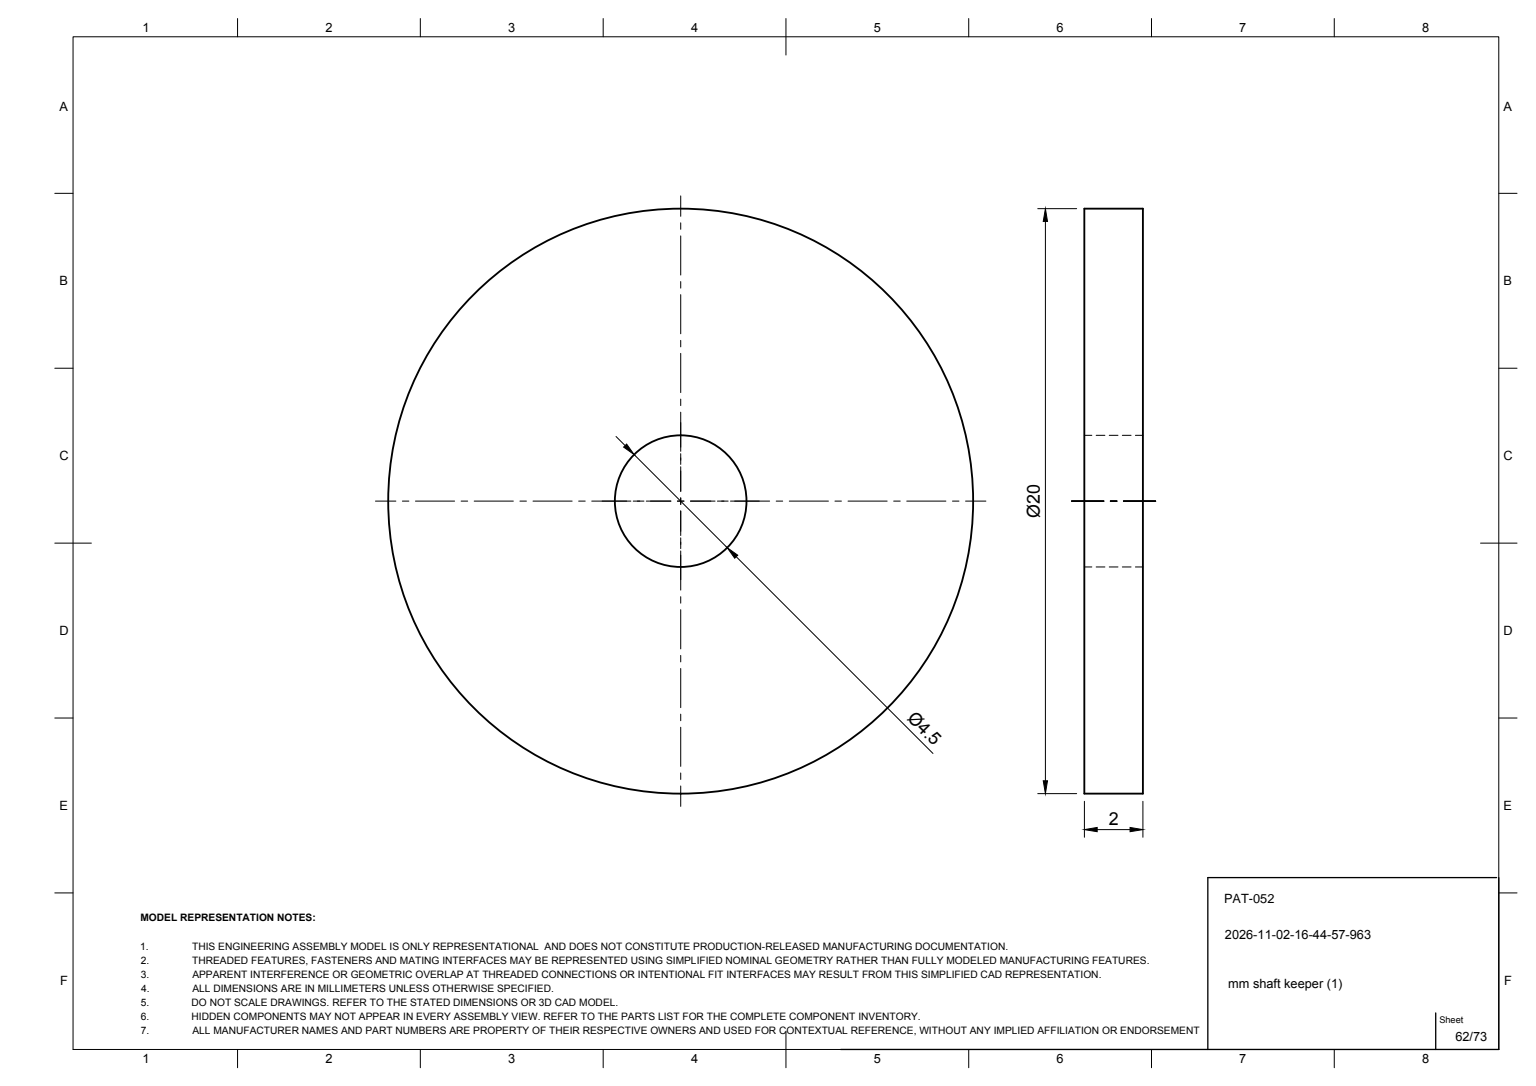
ISO-10303-21;
HEADER;
/* Generated by software containing ST-Developer
 * from STEP Tools, Inc. (www.steptools.com) 
 */

FILE_DESCRIPTION(
/* description */ ('Hand-crank gear train demonstrator'),
/* implementation_level */ '2;1');

FILE_NAME(
/* name */ 'mm shaft keeper (1).step',
/* time_stamp */ '2026-10-28T03:22:13-07:00',
/* author */ (''),
/* organization */ (''),
/* preprocessor_version */ 'ST-DEVELOPER v20.2',
/* originating_system */ 'Autodesk Translation Framework v15.17.0.0',
/* authorisation */ '');

FILE_SCHEMA (('AUTOMOTIVE_DESIGN { 1 0 10303 214 3 1 1 }'));
ENDSEC;

DATA;
#10=MECHANICAL_DESIGN_GEOMETRIC_PRESENTATION_REPRESENTATION('',(#1252),#62758);
#1109=SHAPE_REPRESENTATION_RELATIONSHIP('SRR','None',#63086,#1173);
#1173=ADVANCED_BREP_SHAPE_REPRESENTATION('',(#1327),#62740);
#1252=STYLED_ITEM('',(#63462),#1327);
#1327=MANIFOLD_SOLID_BREP('Body1',#16436);
#1598=FACE_BOUND('',#3889,.T.);
#1599=FACE_BOUND('',#3891,.T.);
#1975=PLANE('',#18269);
#1976=PLANE('',#18270);
#2694=FACE_OUTER_BOUND('',#3886,.T.);
#2695=FACE_OUTER_BOUND('',#3887,.T.);
#2696=FACE_OUTER_BOUND('',#3888,.T.);
#2697=FACE_OUTER_BOUND('',#3890,.T.);
#3886=EDGE_LOOP('',(#13243,#13244,#13245,#13246));
#3887=EDGE_LOOP('',(#13247,#13248,#13249,#13250));
#3888=EDGE_LOOP('',(#13251));
#3889=EDGE_LOOP('',(#13252));
#3890=EDGE_LOOP('',(#13253));
#3891=EDGE_LOOP('',(#13254));
#4978=LINE('',#26767,#6110);
#4979=LINE('',#26773,#6111);
#6110=VECTOR('',#21737,0.225);
#6111=VECTOR('',#21744,1.);
#7018=CIRCLE('',#18264,0.225);
#7019=CIRCLE('',#18265,0.225);
#7020=CIRCLE('',#18267,1.);
#7021=CIRCLE('',#18268,1.);
#8029=VERTEX_POINT('',#26764);
#8030=VERTEX_POINT('',#26766);
#8031=VERTEX_POINT('',#26770);
#8032=VERTEX_POINT('',#26772);
#9873=EDGE_CURVE('',#8029,#8029,#7018,.T.);
#9874=EDGE_CURVE('',#8029,#8030,#4978,.T.);
#9875=EDGE_CURVE('',#8030,#8030,#7019,.T.);
#9876=EDGE_CURVE('',#8031,#8031,#7020,.T.);
#9877=EDGE_CURVE('',#8031,#8032,#4979,.T.);
#9878=EDGE_CURVE('',#8032,#8032,#7021,.T.);
#13243=ORIENTED_EDGE('',*,*,#9873,.F.);
#13244=ORIENTED_EDGE('',*,*,#9874,.T.);
#13245=ORIENTED_EDGE('',*,*,#9875,.T.);
#13246=ORIENTED_EDGE('',*,*,#9874,.F.);
#13247=ORIENTED_EDGE('',*,*,#9876,.F.);
#13248=ORIENTED_EDGE('',*,*,#9877,.T.);
#13249=ORIENTED_EDGE('',*,*,#9878,.T.);
#13250=ORIENTED_EDGE('',*,*,#9877,.F.);
#13251=ORIENTED_EDGE('',*,*,#9876,.T.);
#13252=ORIENTED_EDGE('',*,*,#9873,.T.);
#13253=ORIENTED_EDGE('',*,*,#9878,.F.);
#13254=ORIENTED_EDGE('',*,*,#9875,.F.);
#15342=CYLINDRICAL_SURFACE('',#18263,0.225);
#15343=CYLINDRICAL_SURFACE('',#18266,1.);
#16004=ADVANCED_FACE('',(#2694),#15342,.F.);
#16005=ADVANCED_FACE('',(#2695),#15343,.T.);
#16006=ADVANCED_FACE('',(#2696,#1598),#1975,.T.);
#16007=ADVANCED_FACE('',(#2697,#1599),#1976,.F.);
#16436=CLOSED_SHELL('',(#16004,#16005,#16006,#16007));
#18262=AXIS2_PLACEMENT_3D('',#26762,#21731,#21732);
#18263=AXIS2_PLACEMENT_3D('',#26763,#21733,#21734);
#18264=AXIS2_PLACEMENT_3D('',#26765,#21735,#21736);
#18265=AXIS2_PLACEMENT_3D('',#26768,#21738,#21739);
#18266=AXIS2_PLACEMENT_3D('',#26769,#21740,#21741);
#18267=AXIS2_PLACEMENT_3D('',#26771,#21742,#21743);
#18268=AXIS2_PLACEMENT_3D('',#26774,#21745,#21746);
#18269=AXIS2_PLACEMENT_3D('',#26775,#21747,#21748);
#18270=AXIS2_PLACEMENT_3D('',#26776,#21749,#21750);
#21731=DIRECTION('axis',(0.,0.,1.));
#21732=DIRECTION('refdir',(1.,0.,0.));
#21733=DIRECTION('center_axis',(0.,1.,0.));
#21734=DIRECTION('ref_axis',(1.,0.,0.));
#21735=DIRECTION('center_axis',(0.,-1.,0.));
#21736=DIRECTION('ref_axis',(1.,0.,0.));
#21737=DIRECTION('',(0.,-1.,0.));
#21738=DIRECTION('center_axis',(0.,-1.,0.));
#21739=DIRECTION('ref_axis',(1.,0.,0.));
#21740=DIRECTION('center_axis',(0.,1.,0.));
#21741=DIRECTION('ref_axis',(1.,0.,0.));
#21742=DIRECTION('center_axis',(0.,1.,0.));
#21743=DIRECTION('ref_axis',(1.,0.,0.));
#21744=DIRECTION('',(0.,-1.,0.));
#21745=DIRECTION('center_axis',(0.,1.,0.));
#21746=DIRECTION('ref_axis',(1.,0.,0.));
#21747=DIRECTION('center_axis',(0.,1.,0.));
#21748=DIRECTION('ref_axis',(1.,0.,0.));
#21749=DIRECTION('center_axis',(0.,1.,0.));
#21750=DIRECTION('ref_axis',(1.,0.,0.));
#26762=CARTESIAN_POINT('',(0.,0.,0.));
#26763=CARTESIAN_POINT('Origin',(12.,3.2,9.));
#26764=CARTESIAN_POINT('',(11.775,3.4,9.));
#26765=CARTESIAN_POINT('Origin',(12.,3.4,9.));
#26766=CARTESIAN_POINT('',(11.775,3.2,9.));
#26767=CARTESIAN_POINT('',(11.775,3.2,9.));
#26768=CARTESIAN_POINT('Origin',(12.,3.2,9.));
#26769=CARTESIAN_POINT('Origin',(12.,3.2,9.));
#26770=CARTESIAN_POINT('',(11.,3.4,9.));
#26771=CARTESIAN_POINT('Origin',(12.,3.4,9.));
#26772=CARTESIAN_POINT('',(11.,3.2,9.));
#26773=CARTESIAN_POINT('',(11.,3.2,9.));
#26774=CARTESIAN_POINT('Origin',(12.,3.2,9.));
#26775=CARTESIAN_POINT('Origin',(12.,3.4,9.));
#26776=CARTESIAN_POINT('Origin',(12.,3.2,9.));
#62666=UNCERTAINTY_MEASURE_WITH_UNIT(LENGTH_MEASURE(0.001),#62759,
'DISTANCE_ACCURACY_VALUE',
'Maximum model space distance between geometric entities at asserted c
onnectivities');
#62684=UNCERTAINTY_MEASURE_WITH_UNIT(LENGTH_MEASURE(0.001),#62759,
'DISTANCE_ACCURACY_VALUE',
'Maximum model space distance between geometric entities at asserted c
onnectivities');
#62740=(
GEOMETRIC_REPRESENTATION_CONTEXT(3)
GLOBAL_UNCERTAINTY_ASSIGNED_CONTEXT((#62666))
GLOBAL_UNIT_ASSIGNED_CONTEXT((#62759,#62761,#62762))
REPRESENTATION_CONTEXT('','3D')
);
#62758=(
GEOMETRIC_REPRESENTATION_CONTEXT(3)
GLOBAL_UNCERTAINTY_ASSIGNED_CONTEXT((#62684))
GLOBAL_UNIT_ASSIGNED_CONTEXT((#62759,#62761,#62762))
REPRESENTATION_CONTEXT('','3D')
);
#62759=(
LENGTH_UNIT()
NAMED_UNIT(*)
SI_UNIT(.CENTI.,.METRE.)
);
#62761=(
NAMED_UNIT(*)
PLANE_ANGLE_UNIT()
SI_UNIT($,.RADIAN.)
);
#62762=(
NAMED_UNIT(*)
SI_UNIT($,.STERADIAN.)
SOLID_ANGLE_UNIT()
);
#62818=SHAPE_DEFINITION_REPRESENTATION(#62901,#63086);
#62901=PRODUCT_DEFINITION_SHAPE('',$,#63160);
#63086=SHAPE_REPRESENTATION('',(#18262),#62740);
#63104=PRODUCT_DEFINITION_CONTEXT('part definition',#63325,'design');
#63160=PRODUCT_DEFINITION('mm shaft keeper (1)','mm shaft keeper (1)',#63233,
#63104);
#63233=PRODUCT_DEFINITION_FORMATION('',$,#63382);
#63325=APPLICATION_CONTEXT(
'Core Data for Automotive Mechanical Design Process');
#63326=PRODUCT_CONTEXT('part definition',#63325,'mechanical');
#63382=PRODUCT('mm shaft keeper (1)','mm shaft keeper (1)',
'mm shaft keeper (1)',(#63326));
#63456=COLOUR_RGB('Grey',0.48,0.52,0.57);
#63457=FILL_AREA_STYLE_COLOUR('',#63456);
#63458=FILL_AREA_STYLE('',(#63457));
#63459=SURFACE_STYLE_FILL_AREA(#63458);
#63460=SURFACE_SIDE_STYLE('',(#63459));
#63461=SURFACE_STYLE_USAGE(.BOTH.,#63460);
#63462=PRESENTATION_STYLE_ASSIGNMENT((#63461));
ENDSEC;
END-ISO-10303-21;
